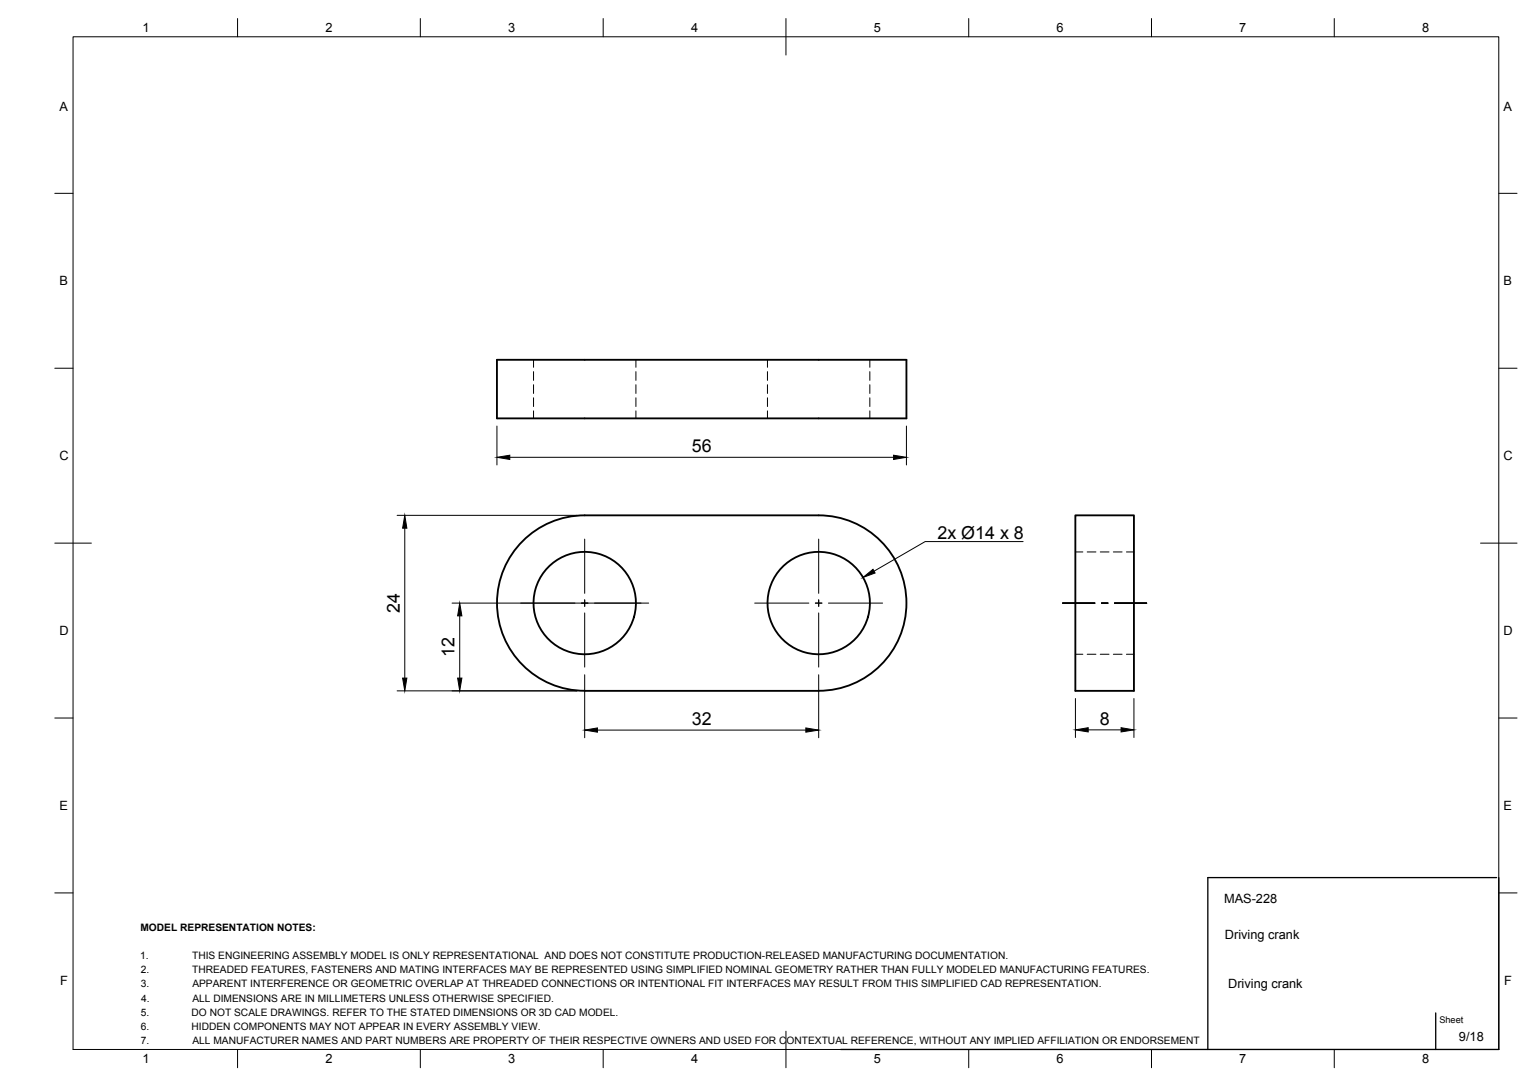
ISO-10303-21;
HEADER;
/* Generated by software containing ST-Developer
 * from STEP Tools, Inc. (www.steptools.com) 
 */

FILE_DESCRIPTION(
/* description */ ('Independent Peaucellier-Lipkin straight-line linkage. Radius arms 100
 mm, inversion-cell links 60 mm, crank radius and fixed-pivot spacing 
32 mm. Inversion constant 6400 mm squared, nominal output straight lin
e X=100 mm. Overhead bearing bridge clears the layered moving links. N
o accuracy or load rating assigned.'),
/* implementation_level */ '2;1');

FILE_NAME(
/* name */ 'Driving crank.step',
/* time_stamp */ '2026-11-09T18:06:16-08:00',
/* author */ (''),
/* organization */ (''),
/* preprocessor_version */ 'ST-DEVELOPER v20.2',
/* originating_system */ 'Autodesk Translation Framework v15.17.0.0',
/* authorisation */ '');

FILE_SCHEMA (('AUTOMOTIVE_DESIGN { 1 0 10303 214 3 1 1 }'));
ENDSEC;

DATA;
#10=MECHANICAL_DESIGN_GEOMETRIC_PRESENTATION_REPRESENTATION('',(#285),#3581);
#251=SHAPE_REPRESENTATION_RELATIONSHIP('SRR','None',#3685,#268);
#268=ADVANCED_BREP_SHAPE_REPRESENTATION('',(#302),#3567);
#285=STYLED_ITEM('',(#3779),#302);
#302=MANIFOLD_SOLID_BREP('Body1',#1871);
#330=FACE_BOUND('',#579,.T.);
#331=FACE_BOUND('',#580,.T.);
#332=FACE_BOUND('',#582,.T.);
#333=FACE_BOUND('',#583,.T.);
#378=PLANE('',#2122);
#379=PLANE('',#2126);
#380=PLANE('',#2130);
#381=PLANE('',#2131);
#447=FACE_OUTER_BOUND('',#572,.T.);
#448=FACE_OUTER_BOUND('',#573,.T.);
#449=FACE_OUTER_BOUND('',#574,.T.);
#450=FACE_OUTER_BOUND('',#575,.T.);
#451=FACE_OUTER_BOUND('',#576,.T.);
#452=FACE_OUTER_BOUND('',#577,.T.);
#453=FACE_OUTER_BOUND('',#578,.T.);
#454=FACE_OUTER_BOUND('',#581,.T.);
#572=EDGE_LOOP('',(#1412,#1413,#1414,#1415));
#573=EDGE_LOOP('',(#1416,#1417,#1418,#1419));
#574=EDGE_LOOP('',(#1420,#1421,#1422,#1423));
#575=EDGE_LOOP('',(#1424,#1425,#1426,#1427));
#576=EDGE_LOOP('',(#1428,#1429,#1430,#1431));
#577=EDGE_LOOP('',(#1432,#1433,#1434,#1435));
#578=EDGE_LOOP('',(#1436,#1437,#1438,#1439));
#579=EDGE_LOOP('',(#1440));
#580=EDGE_LOOP('',(#1441));
#581=EDGE_LOOP('',(#1442,#1443,#1444,#1445));
#582=EDGE_LOOP('',(#1446));
#583=EDGE_LOOP('',(#1447));
#727=LINE('',#3140,#825);
#728=LINE('',#3146,#826);
#729=LINE('',#3151,#827);
#730=LINE('',#3153,#828);
#731=LINE('',#3155,#829);
#732=LINE('',#3156,#830);
#733=LINE('',#3162,#831);
#734=LINE('',#3165,#832);
#735=LINE('',#3167,#833);
#736=LINE('',#3168,#834);
#825=VECTOR('',#2481,7.);
#826=VECTOR('',#2488,7.);
#827=VECTOR('',#2493,10.);
#828=VECTOR('',#2494,10.);
#829=VECTOR('',#2495,10.);
#830=VECTOR('',#2496,10.);
#831=VECTOR('',#2503,10.);
#832=VECTOR('',#2506,10.);
#833=VECTOR('',#2507,10.);
#834=VECTOR('',#2508,10.);
#907=CIRCLE('',#2117,7.);
#908=CIRCLE('',#2118,7.);
#909=CIRCLE('',#2120,7.);
#910=CIRCLE('',#2121,7.);
#911=CIRCLE('',#2124,12.);
#912=CIRCLE('',#2125,12.);
#913=CIRCLE('',#2128,12.);
#914=CIRCLE('',#2129,12.);
#1021=VERTEX_POINT('',#3137);
#1022=VERTEX_POINT('',#3139);
#1023=VERTEX_POINT('',#3143);
#1024=VERTEX_POINT('',#3145);
#1025=VERTEX_POINT('',#3149);
#1026=VERTEX_POINT('',#3150);
#1027=VERTEX_POINT('',#3152);
#1028=VERTEX_POINT('',#3154);
#1029=VERTEX_POINT('',#3158);
#1030=VERTEX_POINT('',#3160);
#1031=VERTEX_POINT('',#3164);
#1032=VERTEX_POINT('',#3166);
#1168=EDGE_CURVE('',#1021,#1021,#907,.T.);
#1169=EDGE_CURVE('',#1021,#1022,#727,.T.);
#1170=EDGE_CURVE('',#1022,#1022,#908,.T.);
#1171=EDGE_CURVE('',#1023,#1023,#909,.T.);
#1172=EDGE_CURVE('',#1023,#1024,#728,.T.);
#1173=EDGE_CURVE('',#1024,#1024,#910,.T.);
#1174=EDGE_CURVE('',#1025,#1026,#729,.T.);
#1175=EDGE_CURVE('',#1026,#1027,#730,.T.);
#1176=EDGE_CURVE('',#1028,#1027,#731,.T.);
#1177=EDGE_CURVE('',#1025,#1028,#732,.T.);
#1178=EDGE_CURVE('',#1029,#1025,#911,.T.);
#1179=EDGE_CURVE('',#1030,#1028,#912,.T.);
#1180=EDGE_CURVE('',#1029,#1030,#733,.T.);
#1181=EDGE_CURVE('',#1031,#1029,#734,.T.);
#1182=EDGE_CURVE('',#1032,#1030,#735,.T.);
#1183=EDGE_CURVE('',#1031,#1032,#736,.T.);
#1184=EDGE_CURVE('',#1026,#1031,#913,.T.);
#1185=EDGE_CURVE('',#1027,#1032,#914,.T.);
#1412=ORIENTED_EDGE('',*,*,#1168,.F.);
#1413=ORIENTED_EDGE('',*,*,#1169,.T.);
#1414=ORIENTED_EDGE('',*,*,#1170,.F.);
#1415=ORIENTED_EDGE('',*,*,#1169,.F.);
#1416=ORIENTED_EDGE('',*,*,#1171,.F.);
#1417=ORIENTED_EDGE('',*,*,#1172,.T.);
#1418=ORIENTED_EDGE('',*,*,#1173,.F.);
#1419=ORIENTED_EDGE('',*,*,#1172,.F.);
#1420=ORIENTED_EDGE('',*,*,#1174,.T.);
#1421=ORIENTED_EDGE('',*,*,#1175,.T.);
#1422=ORIENTED_EDGE('',*,*,#1176,.F.);
#1423=ORIENTED_EDGE('',*,*,#1177,.F.);
#1424=ORIENTED_EDGE('',*,*,#1178,.T.);
#1425=ORIENTED_EDGE('',*,*,#1177,.T.);
#1426=ORIENTED_EDGE('',*,*,#1179,.F.);
#1427=ORIENTED_EDGE('',*,*,#1180,.F.);
#1428=ORIENTED_EDGE('',*,*,#1181,.T.);
#1429=ORIENTED_EDGE('',*,*,#1180,.T.);
#1430=ORIENTED_EDGE('',*,*,#1182,.F.);
#1431=ORIENTED_EDGE('',*,*,#1183,.F.);
#1432=ORIENTED_EDGE('',*,*,#1184,.T.);
#1433=ORIENTED_EDGE('',*,*,#1183,.T.);
#1434=ORIENTED_EDGE('',*,*,#1185,.F.);
#1435=ORIENTED_EDGE('',*,*,#1175,.F.);
#1436=ORIENTED_EDGE('',*,*,#1185,.T.);
#1437=ORIENTED_EDGE('',*,*,#1182,.T.);
#1438=ORIENTED_EDGE('',*,*,#1179,.T.);
#1439=ORIENTED_EDGE('',*,*,#1176,.T.);
#1440=ORIENTED_EDGE('',*,*,#1168,.T.);
#1441=ORIENTED_EDGE('',*,*,#1171,.T.);
#1442=ORIENTED_EDGE('',*,*,#1184,.F.);
#1443=ORIENTED_EDGE('',*,*,#1174,.F.);
#1444=ORIENTED_EDGE('',*,*,#1178,.F.);
#1445=ORIENTED_EDGE('',*,*,#1181,.F.);
#1446=ORIENTED_EDGE('',*,*,#1170,.T.);
#1447=ORIENTED_EDGE('',*,*,#1173,.T.);
#1716=CYLINDRICAL_SURFACE('',#2116,7.);
#1717=CYLINDRICAL_SURFACE('',#2119,7.);
#1718=CYLINDRICAL_SURFACE('',#2123,12.);
#1719=CYLINDRICAL_SURFACE('',#2127,12.);
#1779=ADVANCED_FACE('',(#447),#1716,.F.);
#1780=ADVANCED_FACE('',(#448),#1717,.F.);
#1781=ADVANCED_FACE('',(#449),#378,.T.);
#1782=ADVANCED_FACE('',(#450),#1718,.T.);
#1783=ADVANCED_FACE('',(#451),#379,.T.);
#1784=ADVANCED_FACE('',(#452),#1719,.T.);
#1785=ADVANCED_FACE('',(#453,#330,#331),#380,.T.);
#1786=ADVANCED_FACE('',(#454,#332,#333),#381,.F.);
#1871=CLOSED_SHELL('',(#1779,#1780,#1781,#1782,#1783,#1784,#1785,#1786));
#2115=AXIS2_PLACEMENT_3D('',#3135,#2475,#2476);
#2116=AXIS2_PLACEMENT_3D('',#3136,#2477,#2478);
#2117=AXIS2_PLACEMENT_3D('',#3138,#2479,#2480);
#2118=AXIS2_PLACEMENT_3D('',#3141,#2482,#2483);
#2119=AXIS2_PLACEMENT_3D('',#3142,#2484,#2485);
#2120=AXIS2_PLACEMENT_3D('',#3144,#2486,#2487);
#2121=AXIS2_PLACEMENT_3D('',#3147,#2489,#2490);
#2122=AXIS2_PLACEMENT_3D('',#3148,#2491,#2492);
#2123=AXIS2_PLACEMENT_3D('',#3157,#2497,#2498);
#2124=AXIS2_PLACEMENT_3D('',#3159,#2499,#2500);
#2125=AXIS2_PLACEMENT_3D('',#3161,#2501,#2502);
#2126=AXIS2_PLACEMENT_3D('',#3163,#2504,#2505);
#2127=AXIS2_PLACEMENT_3D('',#3169,#2509,#2510);
#2128=AXIS2_PLACEMENT_3D('',#3170,#2511,#2512);
#2129=AXIS2_PLACEMENT_3D('',#3171,#2513,#2514);
#2130=AXIS2_PLACEMENT_3D('',#3172,#2515,#2516);
#2131=AXIS2_PLACEMENT_3D('',#3173,#2517,#2518);
#2475=DIRECTION('axis',(0.,0.,1.));
#2476=DIRECTION('refdir',(1.,0.,0.));
#2477=DIRECTION('center_axis',(0.,0.,-1.));
#2478=DIRECTION('ref_axis',(1.,0.,0.));
#2479=DIRECTION('center_axis',(0.,0.,-1.));
#2480=DIRECTION('ref_axis',(1.,0.,0.));
#2481=DIRECTION('',(0.,0.,-1.));
#2482=DIRECTION('center_axis',(0.,0.,1.));
#2483=DIRECTION('ref_axis',(1.,0.,0.));
#2484=DIRECTION('center_axis',(0.,0.,-1.));
#2485=DIRECTION('ref_axis',(1.,0.,0.));
#2486=DIRECTION('center_axis',(0.,0.,-1.));
#2487=DIRECTION('ref_axis',(1.,0.,0.));
#2488=DIRECTION('',(0.,0.,-1.));
#2489=DIRECTION('center_axis',(0.,0.,1.));
#2490=DIRECTION('ref_axis',(1.,0.,0.));
#2491=DIRECTION('center_axis',(0.,1.,0.));
#2492=DIRECTION('ref_axis',(-1.,0.,0.));
#2493=DIRECTION('',(-1.,0.,0.));
#2494=DIRECTION('',(0.,0.,1.));
#2495=DIRECTION('',(-1.,0.,0.));
#2496=DIRECTION('',(0.,0.,1.));
#2497=DIRECTION('center_axis',(0.,0.,1.));
#2498=DIRECTION('ref_axis',(0.,-1.,0.));
#2499=DIRECTION('center_axis',(0.,0.,1.));
#2500=DIRECTION('ref_axis',(0.,-1.,0.));
#2501=DIRECTION('center_axis',(0.,0.,1.));
#2502=DIRECTION('ref_axis',(0.,-1.,0.));
#2503=DIRECTION('',(0.,0.,1.));
#2504=DIRECTION('center_axis',(0.,-1.,0.));
#2505=DIRECTION('ref_axis',(1.,0.,0.));
#2506=DIRECTION('',(1.,0.,0.));
#2507=DIRECTION('',(1.,0.,0.));
#2508=DIRECTION('',(0.,0.,1.));
#2509=DIRECTION('center_axis',(0.,0.,1.));
#2510=DIRECTION('ref_axis',(0.,1.,0.));
#2511=DIRECTION('center_axis',(0.,0.,1.));
#2512=DIRECTION('ref_axis',(0.,1.,0.));
#2513=DIRECTION('center_axis',(0.,0.,1.));
#2514=DIRECTION('ref_axis',(0.,1.,0.));
#2515=DIRECTION('center_axis',(0.,0.,1.));
#2516=DIRECTION('ref_axis',(1.,0.,0.));
#2517=DIRECTION('center_axis',(0.,0.,1.));
#2518=DIRECTION('ref_axis',(1.,0.,0.));
#3135=CARTESIAN_POINT('',(0.,0.,0.));
#3136=CARTESIAN_POINT('Origin',(0.,0.,4.));
#3137=CARTESIAN_POINT('',(-7.,8.57252759403147E-16,8.));
#3138=CARTESIAN_POINT('Origin',(0.,0.,8.));
#3139=CARTESIAN_POINT('',(-7.,8.57252759403147E-16,0.));
#3140=CARTESIAN_POINT('',(-7.,8.57252759403147E-16,4.));
#3141=CARTESIAN_POINT('Origin',(0.,0.,0.));
#3142=CARTESIAN_POINT('Origin',(32.,0.,4.));
#3143=CARTESIAN_POINT('',(25.,8.57252759403147E-16,8.));
#3144=CARTESIAN_POINT('Origin',(32.,0.,8.));
#3145=CARTESIAN_POINT('',(25.,8.57252759403147E-16,0.));
#3146=CARTESIAN_POINT('',(25.,8.57252759403147E-16,4.));
#3147=CARTESIAN_POINT('Origin',(32.,0.,0.));
#3148=CARTESIAN_POINT('Origin',(32.,12.,0.));
#3149=CARTESIAN_POINT('',(32.,12.,0.));
#3150=CARTESIAN_POINT('',(0.,12.,0.));
#3151=CARTESIAN_POINT('',(32.,12.,0.));
#3152=CARTESIAN_POINT('',(0.,12.,8.));
#3153=CARTESIAN_POINT('',(0.,12.,0.));
#3154=CARTESIAN_POINT('',(32.,12.,8.));
#3155=CARTESIAN_POINT('',(32.,12.,8.));
#3156=CARTESIAN_POINT('',(32.,12.,0.));
#3157=CARTESIAN_POINT('Origin',(32.,0.,0.));
#3158=CARTESIAN_POINT('',(32.,-12.,0.));
#3159=CARTESIAN_POINT('Origin',(32.,0.,0.));
#3160=CARTESIAN_POINT('',(32.,-12.,8.));
#3161=CARTESIAN_POINT('Origin',(32.,0.,8.));
#3162=CARTESIAN_POINT('',(32.,-12.,0.));
#3163=CARTESIAN_POINT('Origin',(0.,-12.,0.));
#3164=CARTESIAN_POINT('',(-1.46957615897682E-15,-12.,0.));
#3165=CARTESIAN_POINT('',(0.,-12.,0.));
#3166=CARTESIAN_POINT('',(-1.46957615897682E-15,-12.,8.));
#3167=CARTESIAN_POINT('',(0.,-12.,8.));
#3168=CARTESIAN_POINT('',(-1.46957615897682E-15,-12.,0.));
#3169=CARTESIAN_POINT('Origin',(0.,0.,0.));
#3170=CARTESIAN_POINT('Origin',(0.,0.,0.));
#3171=CARTESIAN_POINT('Origin',(0.,0.,8.));
#3172=CARTESIAN_POINT('Origin',(16.,0.,8.));
#3173=CARTESIAN_POINT('Origin',(16.,0.,0.));
#3548=UNCERTAINTY_MEASURE_WITH_UNIT(LENGTH_MEASURE(0.01),#3582,
'DISTANCE_ACCURACY_VALUE',
'Maximum model space distance between geometric entities at asserted c
onnectivities');
#3562=UNCERTAINTY_MEASURE_WITH_UNIT(LENGTH_MEASURE(0.01),#3582,
'DISTANCE_ACCURACY_VALUE',
'Maximum model space distance between geometric entities at asserted c
onnectivities');
#3567=(
GEOMETRIC_REPRESENTATION_CONTEXT(3)
GLOBAL_UNCERTAINTY_ASSIGNED_CONTEXT((#3548))
GLOBAL_UNIT_ASSIGNED_CONTEXT((#3582,#3584,#3585))
REPRESENTATION_CONTEXT('','3D')
);
#3581=(
GEOMETRIC_REPRESENTATION_CONTEXT(3)
GLOBAL_UNCERTAINTY_ASSIGNED_CONTEXT((#3562))
GLOBAL_UNIT_ASSIGNED_CONTEXT((#3582,#3584,#3585))
REPRESENTATION_CONTEXT('','3D')
);
#3582=(
LENGTH_UNIT()
NAMED_UNIT(*)
SI_UNIT(.MILLI.,.METRE.)
);
#3584=(
NAMED_UNIT(*)
PLANE_ANGLE_UNIT()
SI_UNIT($,.RADIAN.)
);
#3585=(
NAMED_UNIT(*)
SI_UNIT($,.STERADIAN.)
SOLID_ANGLE_UNIT()
);
#3590=SHAPE_DEFINITION_REPRESENTATION(#3608,#3685);
#3608=PRODUCT_DEFINITION_SHAPE('',$,#3704);
#3685=SHAPE_REPRESENTATION('',(#2115),#3567);
#3699=PRODUCT_DEFINITION_CONTEXT('part definition',#3755,'design');
#3704=PRODUCT_DEFINITION('Driving crank','Driving crank',#3722,#3699);
#3722=PRODUCT_DEFINITION_FORMATION('',$,#3761);
#3755=APPLICATION_CONTEXT(
'Core Data for Automotive Mechanical Design Process');
#3756=PRODUCT_CONTEXT('part definition',#3755,'mechanical');
#3761=PRODUCT('Driving crank','Driving crank','Driving crank',(#3756));
#3779=PRESENTATION_STYLE_ASSIGNMENT((#3792));
#3792=SURFACE_STYLE_USAGE(.BOTH.,#3805);
#3805=SURFACE_SIDE_STYLE('',(#3818));
#3818=SURFACE_STYLE_FILL_AREA(#3831);
#3831=FILL_AREA_STYLE('Driving crank finish',(#3844));
#3844=FILL_AREA_STYLE_COLOUR('Driving crank finish',#3857);
#3857=COLOUR_RGB('Driving crank finish',0.662745098039216,0.831372549019608,
0.949019607843137);
ENDSEC;
END-ISO-10303-21;
